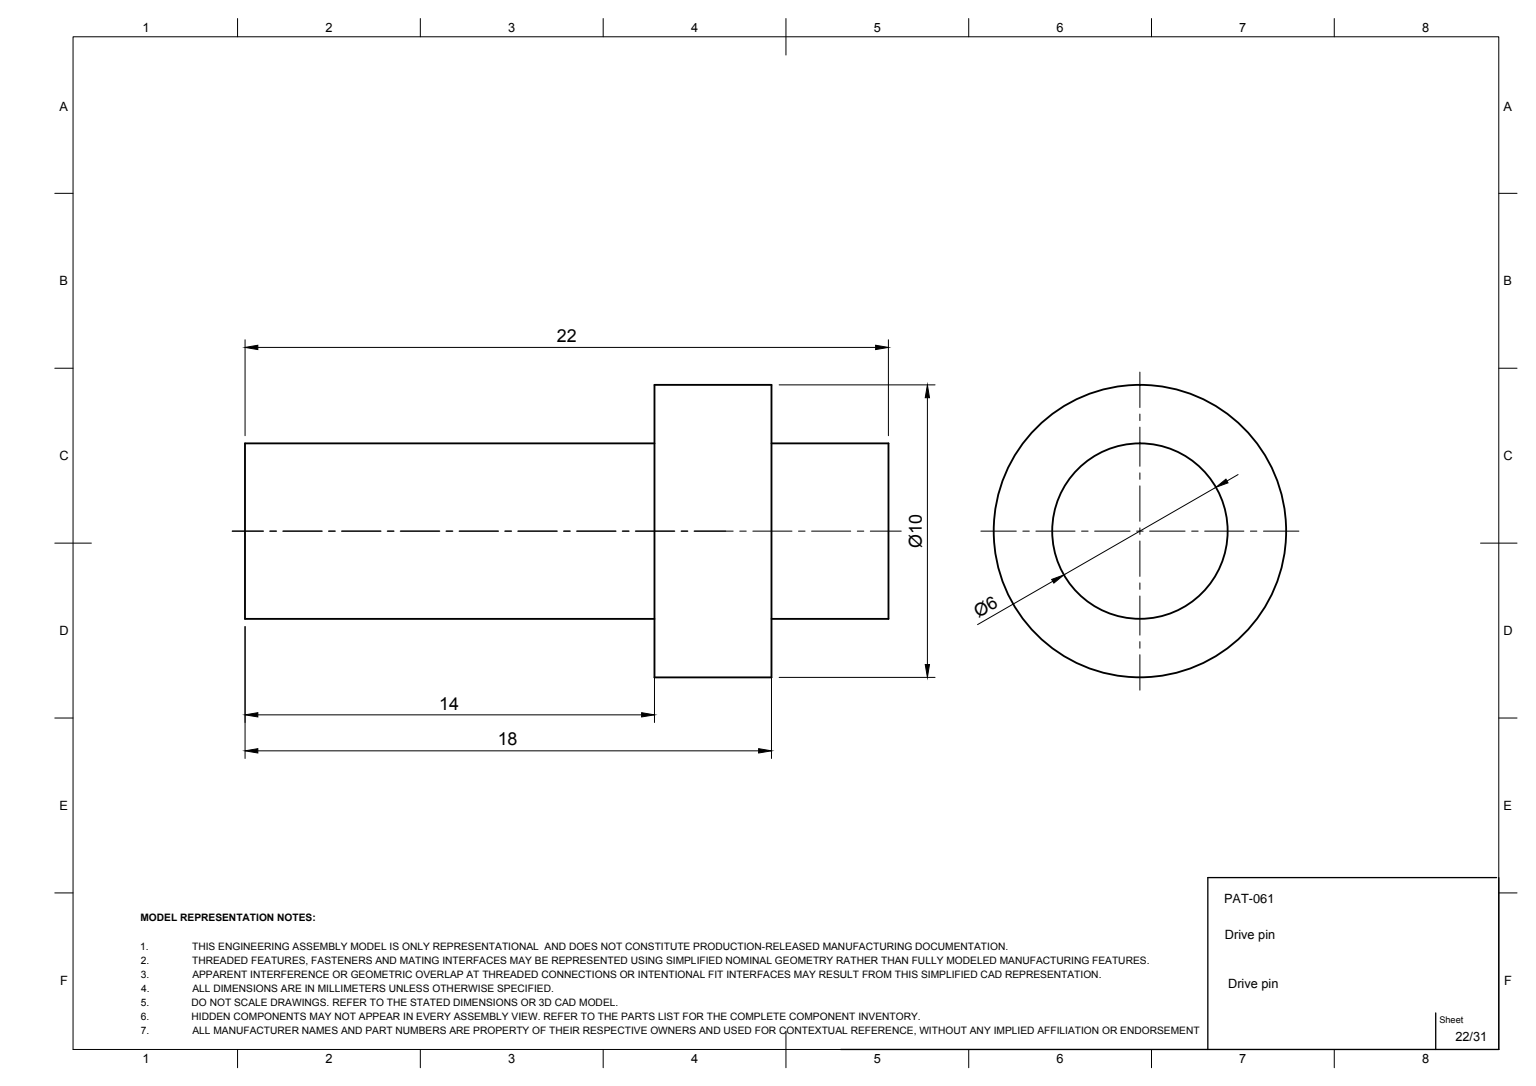
ISO-10303-21;
HEADER;
/* Generated by software containing ST-Developer
 * from STEP Tools, Inc. (www.steptools.com) 
 */

FILE_DESCRIPTION(
/* description */ ('Compact intermittent indexer'),
/* implementation_level */ '2;1');

FILE_NAME(
/* name */ 'Drive pin.step',
/* time_stamp */ '2026-10-29T16:32:17-07:00',
/* author */ (''),
/* organization */ (''),
/* preprocessor_version */ 'ST-DEVELOPER v20.2',
/* originating_system */ 'Autodesk Translation Framework v15.17.0.0',
/* authorisation */ '');

FILE_SCHEMA (('AUTOMOTIVE_DESIGN { 1 0 10303 214 3 1 1 }'));
ENDSEC;

DATA;
#10=MECHANICAL_DESIGN_GEOMETRIC_PRESENTATION_REPRESENTATION('',(#279),#10837);
#223=SHAPE_REPRESENTATION_RELATIONSHIP('SRR','None',#10959,#247);
#247=ADVANCED_BREP_SHAPE_REPRESENTATION('',(#310),#10826);
#279=STYLED_ITEM('',(#11166),#310);
#310=MANIFOLD_SOLID_BREP('Body1',#5652);
#444=FACE_BOUND('',#1282,.T.);
#445=FACE_BOUND('',#1284,.T.);
#575=PLANE('',#6389);
#576=PLANE('',#6392);
#577=PLANE('',#6400);
#578=PLANE('',#6401);
#862=FACE_OUTER_BOUND('',#1281,.T.);
#863=FACE_OUTER_BOUND('',#1283,.T.);
#864=FACE_OUTER_BOUND('',#1285,.T.);
#865=FACE_OUTER_BOUND('',#1286,.T.);
#866=FACE_OUTER_BOUND('',#1287,.T.);
#867=FACE_OUTER_BOUND('',#1288,.T.);
#868=FACE_OUTER_BOUND('',#1289,.T.);
#1281=EDGE_LOOP('',(#4588));
#1282=EDGE_LOOP('',(#4589));
#1283=EDGE_LOOP('',(#4590));
#1284=EDGE_LOOP('',(#4591));
#1285=EDGE_LOOP('',(#4592,#4593,#4594,#4595));
#1286=EDGE_LOOP('',(#4596,#4597,#4598,#4599));
#1287=EDGE_LOOP('',(#4600,#4601,#4602,#4603));
#1288=EDGE_LOOP('',(#4604));
#1289=EDGE_LOOP('',(#4605));
#1615=LINE('',#10012,#1973);
#1616=LINE('',#10015,#1974);
#1617=LINE('',#10020,#1975);
#1973=VECTOR('',#7785,0.5);
#1974=VECTOR('',#7788,0.3);
#1975=VECTOR('',#7795,0.3);
#2375=CIRCLE('',#6390,0.5);
#2376=CIRCLE('',#6391,0.3);
#2377=CIRCLE('',#6393,0.5);
#2378=CIRCLE('',#6394,0.3);
#2379=CIRCLE('',#6397,0.3);
#2380=CIRCLE('',#6399,0.3);
#2783=VERTEX_POINT('',#10002);
#2784=VERTEX_POINT('',#10004);
#2785=VERTEX_POINT('',#10007);
#2786=VERTEX_POINT('',#10009);
#2787=VERTEX_POINT('',#10014);
#2788=VERTEX_POINT('',#10018);
#3416=EDGE_CURVE('',#2783,#2783,#2375,.T.);
#3417=EDGE_CURVE('',#2784,#2784,#2376,.T.);
#3418=EDGE_CURVE('',#2785,#2785,#2377,.T.);
#3419=EDGE_CURVE('',#2786,#2786,#2378,.T.);
#3420=EDGE_CURVE('',#2783,#2785,#1615,.T.);
#3421=EDGE_CURVE('',#2786,#2787,#1616,.T.);
#3422=EDGE_CURVE('',#2787,#2787,#2379,.T.);
#3423=EDGE_CURVE('',#2788,#2788,#2380,.T.);
#3424=EDGE_CURVE('',#2788,#2784,#1617,.T.);
#4588=ORIENTED_EDGE('',*,*,#3416,.T.);
#4589=ORIENTED_EDGE('',*,*,#3417,.F.);
#4590=ORIENTED_EDGE('',*,*,#3418,.F.);
#4591=ORIENTED_EDGE('',*,*,#3419,.F.);
#4592=ORIENTED_EDGE('',*,*,#3416,.F.);
#4593=ORIENTED_EDGE('',*,*,#3420,.T.);
#4594=ORIENTED_EDGE('',*,*,#3418,.T.);
#4595=ORIENTED_EDGE('',*,*,#3420,.F.);
#4596=ORIENTED_EDGE('',*,*,#3419,.T.);
#4597=ORIENTED_EDGE('',*,*,#3421,.T.);
#4598=ORIENTED_EDGE('',*,*,#3422,.T.);
#4599=ORIENTED_EDGE('',*,*,#3421,.F.);
#4600=ORIENTED_EDGE('',*,*,#3423,.F.);
#4601=ORIENTED_EDGE('',*,*,#3424,.T.);
#4602=ORIENTED_EDGE('',*,*,#3417,.T.);
#4603=ORIENTED_EDGE('',*,*,#3424,.F.);
#4604=ORIENTED_EDGE('',*,*,#3423,.T.);
#4605=ORIENTED_EDGE('',*,*,#3422,.F.);
#5252=CYLINDRICAL_SURFACE('',#6395,0.5);
#5253=CYLINDRICAL_SURFACE('',#6396,0.3);
#5254=CYLINDRICAL_SURFACE('',#6398,0.3);
#5505=ADVANCED_FACE('',(#862,#444),#575,.T.);
#5506=ADVANCED_FACE('',(#863,#445),#576,.F.);
#5507=ADVANCED_FACE('',(#864),#5252,.T.);
#5508=ADVANCED_FACE('',(#865),#5253,.T.);
#5509=ADVANCED_FACE('',(#866),#5254,.T.);
#5510=ADVANCED_FACE('',(#867),#577,.T.);
#5511=ADVANCED_FACE('',(#868),#578,.F.);
#5652=CLOSED_SHELL('',(#5505,#5506,#5507,#5508,#5509,#5510,#5511));
#6388=AXIS2_PLACEMENT_3D('',#10000,#7769,#7770);
#6389=AXIS2_PLACEMENT_3D('',#10001,#7771,#7772);
#6390=AXIS2_PLACEMENT_3D('',#10003,#7773,#7774);
#6391=AXIS2_PLACEMENT_3D('',#10005,#7775,#7776);
#6392=AXIS2_PLACEMENT_3D('',#10006,#7777,#7778);
#6393=AXIS2_PLACEMENT_3D('',#10008,#7779,#7780);
#6394=AXIS2_PLACEMENT_3D('',#10010,#7781,#7782);
#6395=AXIS2_PLACEMENT_3D('',#10011,#7783,#7784);
#6396=AXIS2_PLACEMENT_3D('',#10013,#7786,#7787);
#6397=AXIS2_PLACEMENT_3D('',#10016,#7789,#7790);
#6398=AXIS2_PLACEMENT_3D('',#10017,#7791,#7792);
#6399=AXIS2_PLACEMENT_3D('',#10019,#7793,#7794);
#6400=AXIS2_PLACEMENT_3D('',#10021,#7796,#7797);
#6401=AXIS2_PLACEMENT_3D('',#10022,#7798,#7799);
#7769=DIRECTION('axis',(0.,0.,1.));
#7770=DIRECTION('refdir',(1.,0.,0.));
#7771=DIRECTION('center_axis',(0.,0.,1.));
#7772=DIRECTION('ref_axis',(1.,0.,0.));
#7773=DIRECTION('center_axis',(0.,0.,1.));
#7774=DIRECTION('ref_axis',(1.,0.,0.));
#7775=DIRECTION('center_axis',(0.,0.,1.));
#7776=DIRECTION('ref_axis',(1.,0.,0.));
#7777=DIRECTION('center_axis',(0.,0.,1.));
#7778=DIRECTION('ref_axis',(1.,0.,0.));
#7779=DIRECTION('center_axis',(0.,0.,1.));
#7780=DIRECTION('ref_axis',(1.,0.,0.));
#7781=DIRECTION('center_axis',(0.,0.,-1.));
#7782=DIRECTION('ref_axis',(1.,0.,0.));
#7783=DIRECTION('center_axis',(0.,0.,1.));
#7784=DIRECTION('ref_axis',(1.,0.,0.));
#7785=DIRECTION('',(0.,0.,-1.));
#7786=DIRECTION('center_axis',(0.,0.,1.));
#7787=DIRECTION('ref_axis',(1.,0.,0.));
#7788=DIRECTION('',(0.,0.,-1.));
#7789=DIRECTION('center_axis',(0.,0.,1.));
#7790=DIRECTION('ref_axis',(1.,0.,0.));
#7791=DIRECTION('center_axis',(0.,0.,1.));
#7792=DIRECTION('ref_axis',(1.,0.,0.));
#7793=DIRECTION('center_axis',(0.,0.,1.));
#7794=DIRECTION('ref_axis',(1.,0.,0.));
#7795=DIRECTION('',(0.,0.,-1.));
#7796=DIRECTION('center_axis',(0.,0.,1.));
#7797=DIRECTION('ref_axis',(1.,0.,0.));
#7798=DIRECTION('center_axis',(0.,0.,1.));
#7799=DIRECTION('ref_axis',(1.,0.,0.));
#10000=CARTESIAN_POINT('',(0.,0.,0.));
#10001=CARTESIAN_POINT('Origin',(3.,0.,5.6));
#10002=CARTESIAN_POINT('',(2.5,-6.12323399573677E-17,5.6));
#10003=CARTESIAN_POINT('Origin',(3.,0.,5.6));
#10004=CARTESIAN_POINT('',(2.7,-3.67394039744206E-17,5.6));
#10005=CARTESIAN_POINT('Origin',(3.,0.,5.6));
#10006=CARTESIAN_POINT('Origin',(3.,0.,5.2));
#10007=CARTESIAN_POINT('',(2.5,-6.12323399573677E-17,5.2));
#10008=CARTESIAN_POINT('Origin',(3.,0.,5.2));
#10009=CARTESIAN_POINT('',(2.7,3.67394039744206E-17,5.2));
#10010=CARTESIAN_POINT('Origin',(3.,0.,5.2));
#10011=CARTESIAN_POINT('Origin',(3.,0.,5.2));
#10012=CARTESIAN_POINT('',(2.5,-6.12323399573677E-17,5.2));
#10013=CARTESIAN_POINT('Origin',(3.,0.,4.8));
#10014=CARTESIAN_POINT('',(2.7,-3.67394039744206E-17,4.8));
#10015=CARTESIAN_POINT('',(2.7,-3.67394039744206E-17,4.8));
#10016=CARTESIAN_POINT('Origin',(3.,0.,4.8));
#10017=CARTESIAN_POINT('Origin',(3.,0.,4.8));
#10018=CARTESIAN_POINT('',(2.7,-3.67394039744206E-17,7.));
#10019=CARTESIAN_POINT('Origin',(3.,0.,7.));
#10020=CARTESIAN_POINT('',(2.7,-3.67394039744206E-17,4.8));
#10021=CARTESIAN_POINT('Origin',(3.,0.,7.));
#10022=CARTESIAN_POINT('Origin',(3.,0.,4.8));
#10796=UNCERTAINTY_MEASURE_WITH_UNIT(LENGTH_MEASURE(0.001),#10838,
'DISTANCE_ACCURACY_VALUE',
'Maximum model space distance between geometric entities at asserted c
onnectivities');
#10807=UNCERTAINTY_MEASURE_WITH_UNIT(LENGTH_MEASURE(0.001),#10838,
'DISTANCE_ACCURACY_VALUE',
'Maximum model space distance between geometric entities at asserted c
onnectivities');
#10826=(
GEOMETRIC_REPRESENTATION_CONTEXT(3)
GLOBAL_UNCERTAINTY_ASSIGNED_CONTEXT((#10796))
GLOBAL_UNIT_ASSIGNED_CONTEXT((#10838,#10840,#10841))
REPRESENTATION_CONTEXT('','3D')
);
#10837=(
GEOMETRIC_REPRESENTATION_CONTEXT(3)
GLOBAL_UNCERTAINTY_ASSIGNED_CONTEXT((#10807))
GLOBAL_UNIT_ASSIGNED_CONTEXT((#10838,#10840,#10841))
REPRESENTATION_CONTEXT('','3D')
);
#10838=(
LENGTH_UNIT()
NAMED_UNIT(*)
SI_UNIT(.CENTI.,.METRE.)
);
#10840=(
NAMED_UNIT(*)
PLANE_ANGLE_UNIT()
SI_UNIT($,.RADIAN.)
);
#10841=(
NAMED_UNIT(*)
SI_UNIT($,.STERADIAN.)
SOLID_ANGLE_UNIT()
);
#10860=SHAPE_DEFINITION_REPRESENTATION(#10894,#10959);
#10894=PRODUCT_DEFINITION_SHAPE('',$,#10989);
#10959=SHAPE_REPRESENTATION('',(#6388),#10826);
#10970=PRODUCT_DEFINITION_CONTEXT('part definition',#11059,'design');
#10989=PRODUCT_DEFINITION('Drive pin','Drive pin',#11018,#10970);
#11018=PRODUCT_DEFINITION_FORMATION('',$,#11079);
#11059=APPLICATION_CONTEXT(
'Core Data for Automotive Mechanical Design Process');
#11060=PRODUCT_CONTEXT('part definition',#11059,'mechanical');
#11079=PRODUCT('Drive pin','Drive pin','Drive pin',(#11060));
#11160=COLOUR_RGB('Grey',0.48,0.52,0.57);
#11161=FILL_AREA_STYLE_COLOUR('',#11160);
#11162=FILL_AREA_STYLE('',(#11161));
#11163=SURFACE_STYLE_FILL_AREA(#11162);
#11164=SURFACE_SIDE_STYLE('',(#11163));
#11165=SURFACE_STYLE_USAGE(.BOTH.,#11164);
#11166=PRESENTATION_STYLE_ASSIGNMENT((#11165));
ENDSEC;
END-ISO-10303-21;
